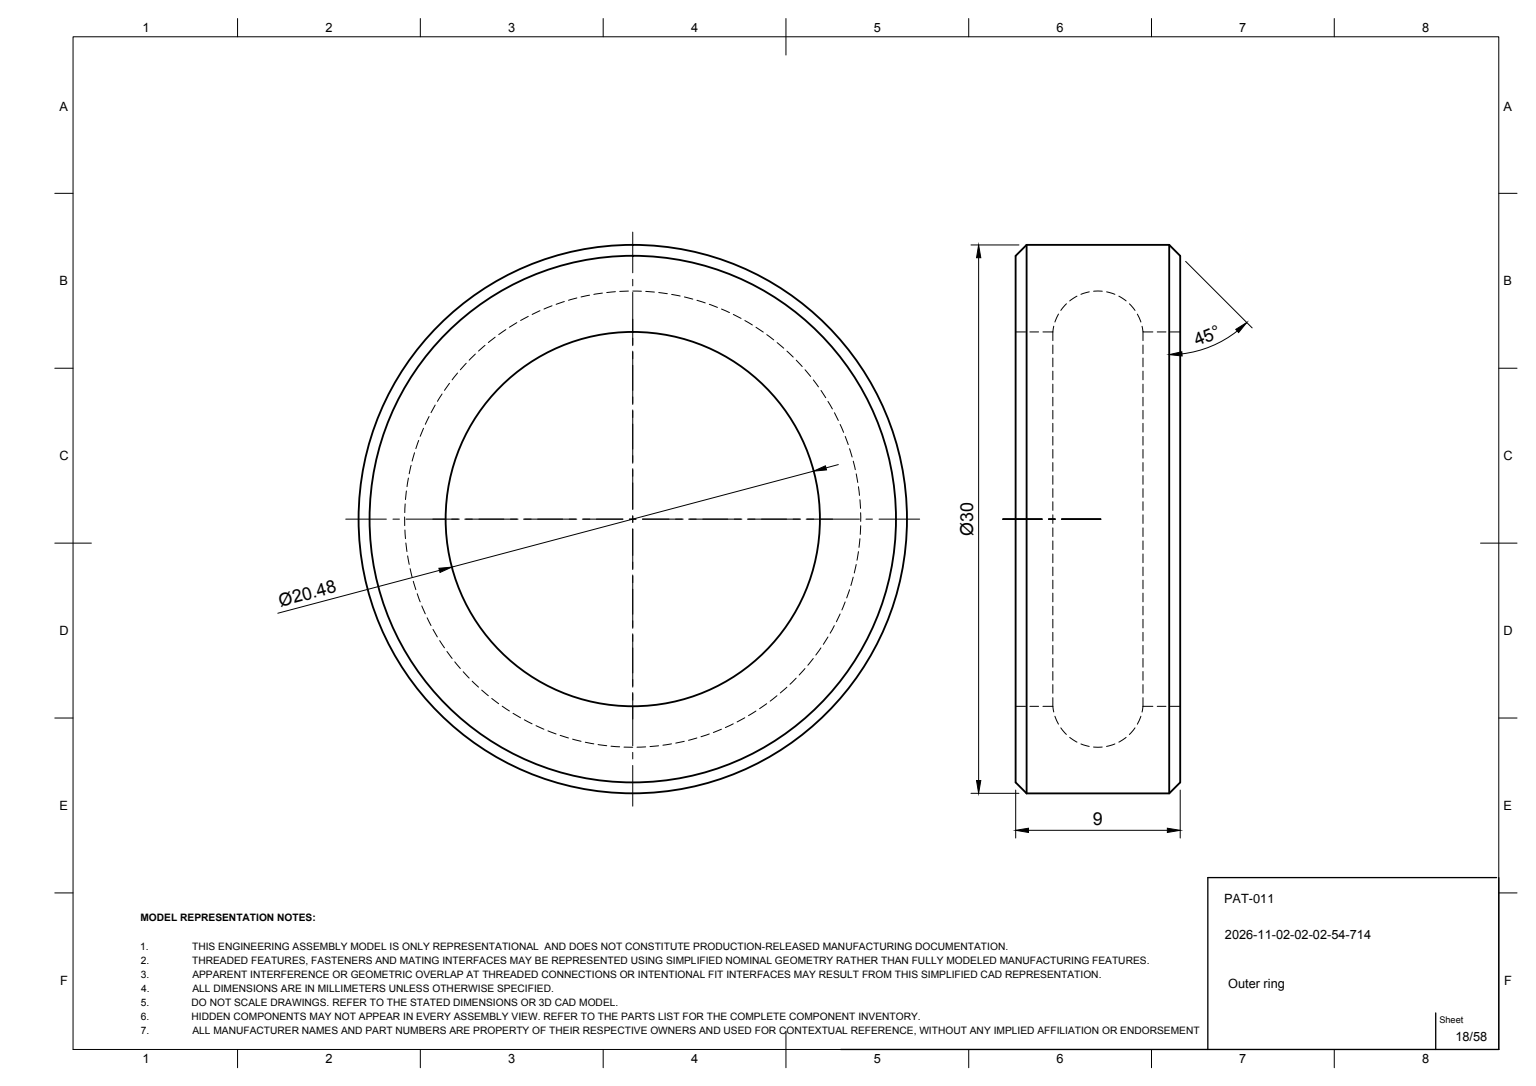
ISO-10303-21;
HEADER;
/* Generated by software containing ST-Developer
 * from STEP Tools, Inc. (www.steptools.com) 
 */

FILE_DESCRIPTION(
/* description */ ('Belt tension measurement rig'),
/* implementation_level */ '2;1');

FILE_NAME(
/* name */ 'Outer ring.step',
/* time_stamp */ '2026-10-28T03:24:44-07:00',
/* author */ (''),
/* organization */ (''),
/* preprocessor_version */ 'ST-DEVELOPER v20.2',
/* originating_system */ 'Autodesk Translation Framework v15.17.0.0',
/* authorisation */ '');

FILE_SCHEMA (('AUTOMOTIVE_DESIGN { 1 0 10303 214 3 1 1 }'));
ENDSEC;

DATA;
#10=MECHANICAL_DESIGN_GEOMETRIC_PRESENTATION_REPRESENTATION('',(#707),#23587);
#469=CONICAL_SURFACE('',#13254,1.47,0.785398163397449);
#470=CONICAL_SURFACE('',#13258,1.47,0.785398163397449);
#488=TOROIDAL_SURFACE('',#13243,1.,0.247676);
#597=SHAPE_REPRESENTATION_RELATIONSHIP('SRR','None',#23843,#652);
#652=ADVANCED_BREP_SHAPE_REPRESENTATION('',(#777),#23541);
#707=STYLED_ITEM('',(#24211),#777);
#777=MANIFOLD_SOLID_BREP('Body1',#12212);
#909=FACE_BOUND('',#2324,.T.);
#910=FACE_BOUND('',#2329,.T.);
#1140=PLANE('',#13251);
#1141=PLANE('',#13260);
#1537=FACE_OUTER_BOUND('',#2321,.T.);
#1538=FACE_OUTER_BOUND('',#2322,.T.);
#1539=FACE_OUTER_BOUND('',#2323,.T.);
#1540=FACE_OUTER_BOUND('',#2325,.T.);
#1541=FACE_OUTER_BOUND('',#2326,.T.);
#1542=FACE_OUTER_BOUND('',#2327,.T.);
#1543=FACE_OUTER_BOUND('',#2328,.T.);
#1544=FACE_OUTER_BOUND('',#2330,.T.);
#2321=EDGE_LOOP('',(#8716,#8717,#8718,#8719,#8720,#8721));
#2322=EDGE_LOOP('',(#8722,#8723,#8724,#8725,#8726));
#2323=EDGE_LOOP('',(#8727));
#2324=EDGE_LOOP('',(#8728));
#2325=EDGE_LOOP('',(#8729,#8730,#8731,#8732));
#2326=EDGE_LOOP('',(#8733,#8734,#8735,#8736));
#2327=EDGE_LOOP('',(#8737,#8738,#8739,#8740));
#2328=EDGE_LOOP('',(#8741));
#2329=EDGE_LOOP('',(#8742));
#2330=EDGE_LOOP('',(#8743,#8744,#8745,#8746,#8747));
#3190=LINE('',#19484,#3941);
#3191=LINE('',#19493,#3942);
#3192=LINE('',#19497,#3943);
#3193=LINE('',#19501,#3944);
#3194=LINE('',#19504,#3945);
#3941=VECTOR('',#15489,1.023815);
#3942=VECTOR('',#15500,1.47);
#3943=VECTOR('',#15505,1.5);
#3944=VECTOR('',#15510,1.47);
#3945=VECTOR('',#15515,1.023815);
#4633=CIRCLE('',#13244,1.023815);
#4634=CIRCLE('',#13245,1.023815);
#4635=CIRCLE('',#13246,0.247676);
#4636=CIRCLE('',#13247,1.023815);
#4637=CIRCLE('',#13248,1.023815);
#4638=CIRCLE('',#13250,1.023815);
#4639=CIRCLE('',#13252,1.44);
#4640=CIRCLE('',#13253,1.023815);
#4641=CIRCLE('',#13255,1.5);
#4642=CIRCLE('',#13257,1.5);
#4643=CIRCLE('',#13259,1.44);
#5494=VERTEX_POINT('',#19472);
#5495=VERTEX_POINT('',#19473);
#5496=VERTEX_POINT('',#19476);
#5497=VERTEX_POINT('',#19478);
#5498=VERTEX_POINT('',#19482);
#5499=VERTEX_POINT('',#19486);
#5500=VERTEX_POINT('',#19488);
#5501=VERTEX_POINT('',#19491);
#5502=VERTEX_POINT('',#19495);
#5503=VERTEX_POINT('',#19499);
#6717=EDGE_CURVE('',#5494,#5495,#4633,.T.);
#6718=EDGE_CURVE('',#5495,#5494,#4634,.T.);
#6719=EDGE_CURVE('',#5495,#5496,#4635,.T.);
#6720=EDGE_CURVE('',#5497,#5496,#4636,.T.);
#6721=EDGE_CURVE('',#5496,#5497,#4637,.T.);
#6722=EDGE_CURVE('',#5498,#5498,#4638,.T.);
#6723=EDGE_CURVE('',#5498,#5497,#3190,.T.);
#6724=EDGE_CURVE('',#5499,#5499,#4639,.T.);
#6725=EDGE_CURVE('',#5500,#5500,#4640,.T.);
#6726=EDGE_CURVE('',#5501,#5501,#4641,.T.);
#6727=EDGE_CURVE('',#5501,#5499,#3191,.T.);
#6728=EDGE_CURVE('',#5502,#5502,#4642,.T.);
#6729=EDGE_CURVE('',#5502,#5501,#3192,.T.);
#6730=EDGE_CURVE('',#5503,#5503,#4643,.T.);
#6731=EDGE_CURVE('',#5503,#5502,#3193,.T.);
#6732=EDGE_CURVE('',#5494,#5500,#3194,.T.);
#8716=ORIENTED_EDGE('',*,*,#6717,.F.);
#8717=ORIENTED_EDGE('',*,*,#6718,.F.);
#8718=ORIENTED_EDGE('',*,*,#6719,.T.);
#8719=ORIENTED_EDGE('',*,*,#6720,.F.);
#8720=ORIENTED_EDGE('',*,*,#6721,.F.);
#8721=ORIENTED_EDGE('',*,*,#6719,.F.);
#8722=ORIENTED_EDGE('',*,*,#6722,.T.);
#8723=ORIENTED_EDGE('',*,*,#6723,.T.);
#8724=ORIENTED_EDGE('',*,*,#6720,.T.);
#8725=ORIENTED_EDGE('',*,*,#6721,.T.);
#8726=ORIENTED_EDGE('',*,*,#6723,.F.);
#8727=ORIENTED_EDGE('',*,*,#6724,.F.);
#8728=ORIENTED_EDGE('',*,*,#6725,.T.);
#8729=ORIENTED_EDGE('',*,*,#6726,.F.);
#8730=ORIENTED_EDGE('',*,*,#6727,.T.);
#8731=ORIENTED_EDGE('',*,*,#6724,.T.);
#8732=ORIENTED_EDGE('',*,*,#6727,.F.);
#8733=ORIENTED_EDGE('',*,*,#6728,.F.);
#8734=ORIENTED_EDGE('',*,*,#6729,.T.);
#8735=ORIENTED_EDGE('',*,*,#6726,.T.);
#8736=ORIENTED_EDGE('',*,*,#6729,.F.);
#8737=ORIENTED_EDGE('',*,*,#6730,.F.);
#8738=ORIENTED_EDGE('',*,*,#6731,.T.);
#8739=ORIENTED_EDGE('',*,*,#6728,.T.);
#8740=ORIENTED_EDGE('',*,*,#6731,.F.);
#8741=ORIENTED_EDGE('',*,*,#6730,.T.);
#8742=ORIENTED_EDGE('',*,*,#6722,.F.);
#8743=ORIENTED_EDGE('',*,*,#6717,.T.);
#8744=ORIENTED_EDGE('',*,*,#6718,.T.);
#8745=ORIENTED_EDGE('',*,*,#6732,.T.);
#8746=ORIENTED_EDGE('',*,*,#6725,.F.);
#8747=ORIENTED_EDGE('',*,*,#6732,.F.);
#11237=CYLINDRICAL_SURFACE('',#13249,1.023815);
#11238=CYLINDRICAL_SURFACE('',#13256,1.5);
#11239=CYLINDRICAL_SURFACE('',#13261,1.023815);
#11678=ADVANCED_FACE('',(#1537),#488,.F.);
#11679=ADVANCED_FACE('',(#1538),#11237,.F.);
#11680=ADVANCED_FACE('',(#1539,#909),#1140,.T.);
#11681=ADVANCED_FACE('',(#1540),#469,.T.);
#11682=ADVANCED_FACE('',(#1541),#11238,.T.);
#11683=ADVANCED_FACE('',(#1542),#470,.T.);
#11684=ADVANCED_FACE('',(#1543,#910),#1141,.T.);
#11685=ADVANCED_FACE('',(#1544),#11239,.F.);
#12212=CLOSED_SHELL('',(#11678,#11679,#11680,#11681,#11682,#11683,#11684,
#11685));
#13242=AXIS2_PLACEMENT_3D('',#19470,#15471,#15472);
#13243=AXIS2_PLACEMENT_3D('',#19471,#15473,#15474);
#13244=AXIS2_PLACEMENT_3D('',#19474,#15475,#15476);
#13245=AXIS2_PLACEMENT_3D('',#19475,#15477,#15478);
#13246=AXIS2_PLACEMENT_3D('',#19477,#15479,#15480);
#13247=AXIS2_PLACEMENT_3D('',#19479,#15481,#15482);
#13248=AXIS2_PLACEMENT_3D('',#19480,#15483,#15484);
#13249=AXIS2_PLACEMENT_3D('',#19481,#15485,#15486);
#13250=AXIS2_PLACEMENT_3D('',#19483,#15487,#15488);
#13251=AXIS2_PLACEMENT_3D('',#19485,#15490,#15491);
#13252=AXIS2_PLACEMENT_3D('',#19487,#15492,#15493);
#13253=AXIS2_PLACEMENT_3D('',#19489,#15494,#15495);
#13254=AXIS2_PLACEMENT_3D('',#19490,#15496,#15497);
#13255=AXIS2_PLACEMENT_3D('',#19492,#15498,#15499);
#13256=AXIS2_PLACEMENT_3D('',#19494,#15501,#15502);
#13257=AXIS2_PLACEMENT_3D('',#19496,#15503,#15504);
#13258=AXIS2_PLACEMENT_3D('',#19498,#15506,#15507);
#13259=AXIS2_PLACEMENT_3D('',#19500,#15508,#15509);
#13260=AXIS2_PLACEMENT_3D('',#19502,#15511,#15512);
#13261=AXIS2_PLACEMENT_3D('',#19503,#15513,#15514);
#15471=DIRECTION('axis',(0.,0.,1.));
#15472=DIRECTION('refdir',(1.,0.,0.));
#15473=DIRECTION('center_axis',(0.,-1.,0.));
#15474=DIRECTION('ref_axis',(0.,0.,-1.));
#15475=DIRECTION('center_axis',(0.,-1.,0.));
#15476=DIRECTION('ref_axis',(1.,0.,0.));
#15477=DIRECTION('center_axis',(0.,-1.,0.));
#15478=DIRECTION('ref_axis',(1.,0.,0.));
#15479=DIRECTION('center_axis',(1.,0.,1.22464679914735E-16));
#15480=DIRECTION('ref_axis',(-1.22464679914735E-16,0.,1.));
#15481=DIRECTION('center_axis',(0.,1.,0.));
#15482=DIRECTION('ref_axis',(1.,0.,0.));
#15483=DIRECTION('center_axis',(0.,1.,0.));
#15484=DIRECTION('ref_axis',(1.,0.,0.));
#15485=DIRECTION('center_axis',(0.,-1.,0.));
#15486=DIRECTION('ref_axis',(1.,0.,0.));
#15487=DIRECTION('center_axis',(0.,-1.,0.));
#15488=DIRECTION('ref_axis',(1.,0.,0.));
#15489=DIRECTION('',(0.,1.,0.));
#15490=DIRECTION('center_axis',(0.,1.,0.));
#15491=DIRECTION('ref_axis',(0.,0.,1.));
#15492=DIRECTION('center_axis',(0.,-1.,0.));
#15493=DIRECTION('ref_axis',(1.,0.,0.));
#15494=DIRECTION('center_axis',(0.,-1.,0.));
#15495=DIRECTION('ref_axis',(1.,0.,0.));
#15496=DIRECTION('center_axis',(0.,-1.,0.));
#15497=DIRECTION('ref_axis',(1.,0.,0.));
#15498=DIRECTION('center_axis',(0.,-1.,0.));
#15499=DIRECTION('ref_axis',(1.,0.,0.));
#15500=DIRECTION('',(0.707106781186548,0.707106781186547,8.65956056235494E-17));
#15501=DIRECTION('center_axis',(0.,-1.,0.));
#15502=DIRECTION('ref_axis',(1.,0.,0.));
#15503=DIRECTION('center_axis',(0.,-1.,0.));
#15504=DIRECTION('ref_axis',(1.,0.,0.));
#15505=DIRECTION('',(0.,1.,0.));
#15506=DIRECTION('center_axis',(0.,1.,0.));
#15507=DIRECTION('ref_axis',(1.,0.,0.));
#15508=DIRECTION('center_axis',(0.,-1.,0.));
#15509=DIRECTION('ref_axis',(1.,0.,0.));
#15510=DIRECTION('',(-0.707106781186548,0.707106781186547,-8.65956056235494E-17));
#15511=DIRECTION('center_axis',(0.,-1.,0.));
#15512=DIRECTION('ref_axis',(0.,0.,-1.));
#15513=DIRECTION('center_axis',(0.,-1.,0.));
#15514=DIRECTION('ref_axis',(1.,0.,0.));
#15515=DIRECTION('',(0.,1.,0.));
#19470=CARTESIAN_POINT('',(0.,0.,0.));
#19471=CARTESIAN_POINT('Origin',(0.,0.,0.));
#19472=CARTESIAN_POINT('',(-1.023815,0.246528389340863,-1.25381176266905E-16));
#19473=CARTESIAN_POINT('',(-1.25381176266905E-16,0.246528389340863,1.023815));
#19474=CARTESIAN_POINT('Origin',(0.,0.246528389340863,0.));
#19475=CARTESIAN_POINT('Origin',(0.,0.246528389340863,0.));
#19476=CARTESIAN_POINT('',(-1.25381176266905E-16,-0.246528389340863,1.023815));
#19477=CARTESIAN_POINT('Origin',(-1.22464679914735E-16,0.,1.));
#19478=CARTESIAN_POINT('',(-1.023815,-0.246528389340863,1.25381176266905E-16));
#19479=CARTESIAN_POINT('Origin',(0.,-0.246528389340863,0.));
#19480=CARTESIAN_POINT('Origin',(0.,-0.246528389340863,0.));
#19481=CARTESIAN_POINT('Origin',(0.,0.,0.));
#19482=CARTESIAN_POINT('',(-1.023815,-0.45,-1.25381176266905E-16));
#19483=CARTESIAN_POINT('Origin',(0.,-0.45,0.));
#19484=CARTESIAN_POINT('',(-1.023815,0.,-1.25381176266905E-16));
#19485=CARTESIAN_POINT('Origin',(1.44,0.45,0.));
#19486=CARTESIAN_POINT('',(-1.44,0.45,-1.76349139077219E-16));
#19487=CARTESIAN_POINT('Origin',(0.,0.45,0.));
#19488=CARTESIAN_POINT('',(-1.023815,0.45,-1.25381176266905E-16));
#19489=CARTESIAN_POINT('Origin',(0.,0.45,0.));
#19490=CARTESIAN_POINT('Origin',(0.,0.42,0.));
#19491=CARTESIAN_POINT('',(-1.5,0.39,-1.83697019872103E-16));
#19492=CARTESIAN_POINT('Origin',(0.,0.39,0.));
#19493=CARTESIAN_POINT('',(-1.47,0.42,-1.80023079474661E-16));
#19494=CARTESIAN_POINT('Origin',(0.,0.,0.));
#19495=CARTESIAN_POINT('',(-1.5,-0.39,-1.83697019872103E-16));
#19496=CARTESIAN_POINT('Origin',(0.,-0.39,0.));
#19497=CARTESIAN_POINT('',(-1.5,0.,-1.83697019872103E-16));
#19498=CARTESIAN_POINT('Origin',(0.,-0.42,0.));
#19499=CARTESIAN_POINT('',(-1.44,-0.45,-1.76349139077219E-16));
#19500=CARTESIAN_POINT('Origin',(0.,-0.45,0.));
#19501=CARTESIAN_POINT('',(-1.47,-0.42,-1.80023079474661E-16));
#19502=CARTESIAN_POINT('Origin',(1.023815,-0.45,0.));
#19503=CARTESIAN_POINT('Origin',(0.,0.,0.));
#19504=CARTESIAN_POINT('',(-1.023815,0.,-1.25381176266905E-16));
#23476=UNCERTAINTY_MEASURE_WITH_UNIT(LENGTH_MEASURE(0.001),#23588,
'DISTANCE_ACCURACY_VALUE',
'Maximum model space distance between geometric entities at asserted c
onnectivities');
#23522=UNCERTAINTY_MEASURE_WITH_UNIT(LENGTH_MEASURE(0.001),#23588,
'DISTANCE_ACCURACY_VALUE',
'Maximum model space distance between geometric entities at asserted c
onnectivities');
#23541=(
GEOMETRIC_REPRESENTATION_CONTEXT(3)
GLOBAL_UNCERTAINTY_ASSIGNED_CONTEXT((#23476))
GLOBAL_UNIT_ASSIGNED_CONTEXT((#23588,#23590,#23591))
REPRESENTATION_CONTEXT('','3D')
);
#23587=(
GEOMETRIC_REPRESENTATION_CONTEXT(3)
GLOBAL_UNCERTAINTY_ASSIGNED_CONTEXT((#23522))
GLOBAL_UNIT_ASSIGNED_CONTEXT((#23588,#23590,#23591))
REPRESENTATION_CONTEXT('','3D')
);
#23588=(
LENGTH_UNIT()
NAMED_UNIT(*)
SI_UNIT(.CENTI.,.METRE.)
);
#23590=(
NAMED_UNIT(*)
PLANE_ANGLE_UNIT()
SI_UNIT($,.RADIAN.)
);
#23591=(
NAMED_UNIT(*)
SI_UNIT($,.STERADIAN.)
SOLID_ANGLE_UNIT()
);
#23610=SHAPE_DEFINITION_REPRESENTATION(#23674,#23843);
#23674=PRODUCT_DEFINITION_SHAPE('',$,#23908);
#23843=SHAPE_REPRESENTATION('',(#13242),#23541);
#23889=PRODUCT_DEFINITION_CONTEXT('part definition',#24083,'design');
#23908=PRODUCT_DEFINITION('Outer ring','Outer ring',#23972,#23889);
#23972=PRODUCT_DEFINITION_FORMATION('',$,#24103);
#24083=APPLICATION_CONTEXT(
'Core Data for Automotive Mechanical Design Process');
#24084=PRODUCT_CONTEXT('part definition',#24083,'mechanical');
#24103=PRODUCT('Outer ring','Outer ring','Outer ring',(#24084));
#24205=COLOUR_RGB('Grey',0.48,0.52,0.57);
#24206=FILL_AREA_STYLE_COLOUR('',#24205);
#24207=FILL_AREA_STYLE('',(#24206));
#24208=SURFACE_STYLE_FILL_AREA(#24207);
#24209=SURFACE_SIDE_STYLE('',(#24208));
#24210=SURFACE_STYLE_USAGE(.BOTH.,#24209);
#24211=PRESENTATION_STYLE_ASSIGNMENT((#24210));
ENDSEC;
END-ISO-10303-21;
